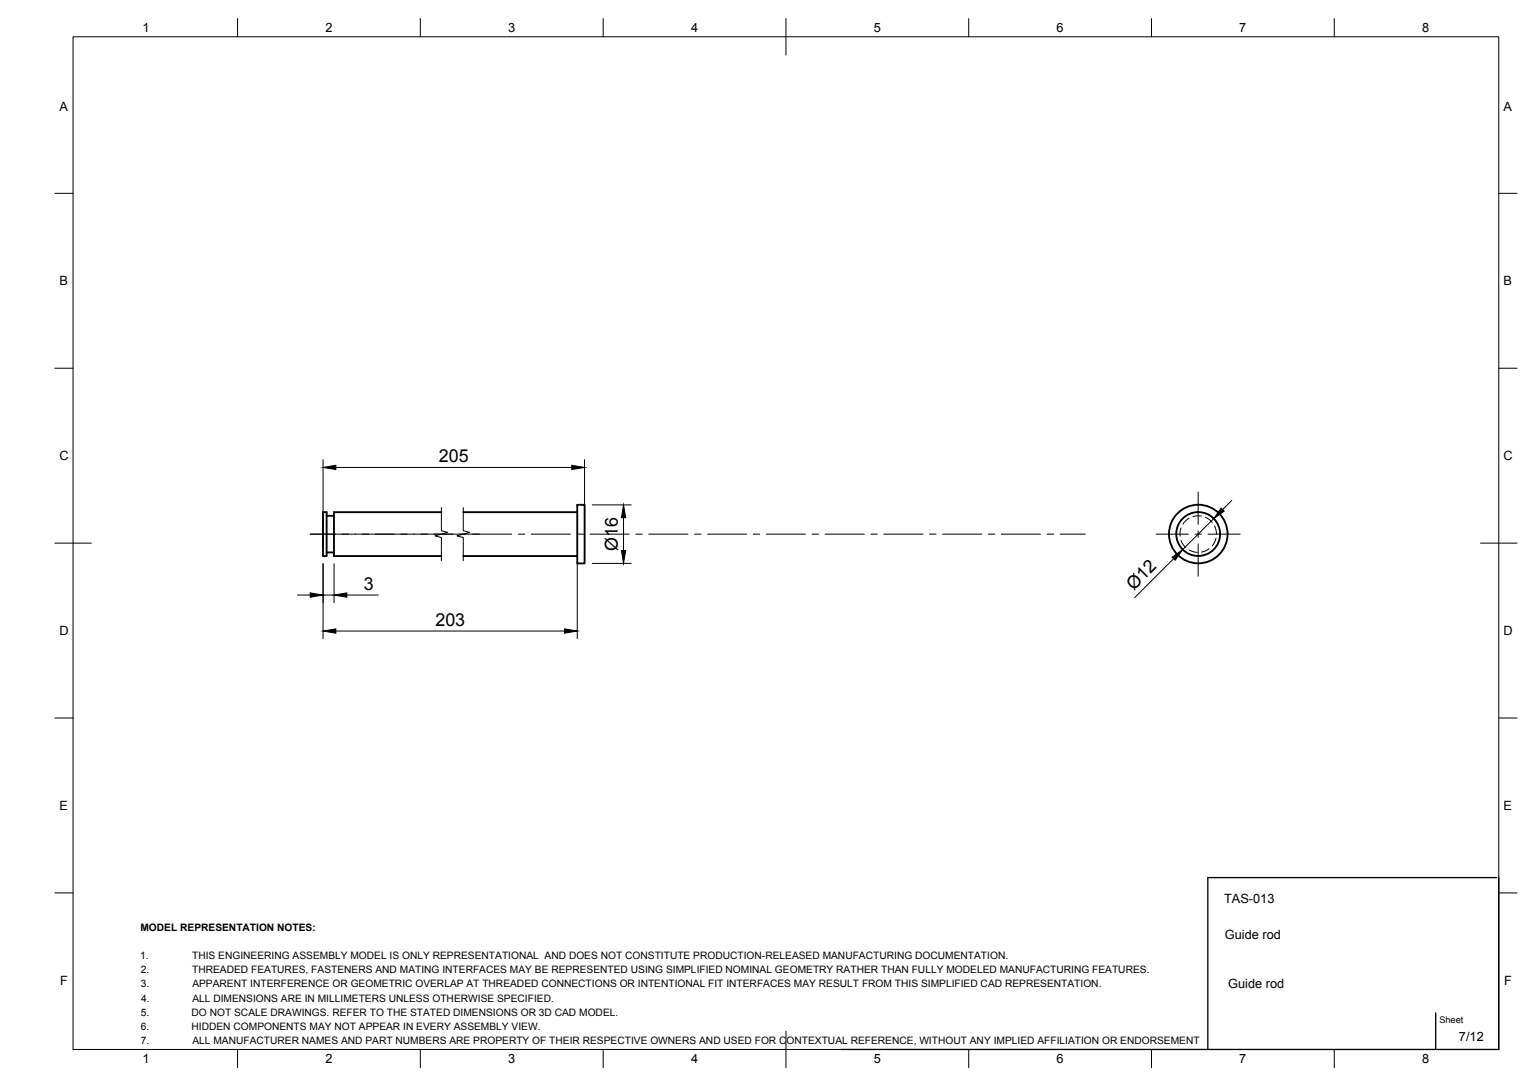
ISO-10303-21;
HEADER;
/* Generated by software containing ST-Developer
 * from STEP Tools, Inc. (www.steptools.com) 
 */

FILE_DESCRIPTION(
/* description */ (
'Independent guided parallel-jaw bracket clamp. Two12mm guide rods, re
placeable bronze sleeves, captured swiveling spindle, replaceable jaw 
pads and modeled M16x2 screw. Native slider/revolute joints linked2mm 
per revolution. Nominal opening0..122 with initial28mm. Base and two i
dentical supports welded. Standard fits, weld details and clamp load r
equire engineering selection.'),
/* implementation_level */ '2;1');

FILE_NAME(
/* name */ 'Guide rod.step',
/* time_stamp */ '2026-11-14T09:15:44-08:00',
/* author */ (''),
/* organization */ (''),
/* preprocessor_version */ 'ST-DEVELOPER v20.2',
/* originating_system */ 'Autodesk Translation Framework v15.17.0.0',
/* authorisation */ '');

FILE_SCHEMA (('AUTOMOTIVE_DESIGN { 1 0 10303 214 3 1 1 }'));
ENDSEC;

DATA;
#10=MECHANICAL_DESIGN_GEOMETRIC_PRESENTATION_REPRESENTATION('',(#922),#105806);
#898=SHAPE_REPRESENTATION_RELATIONSHIP('SRR','None',#105866,#910);
#910=ADVANCED_BREP_SHAPE_REPRESENTATION('',(#934),#105801);
#922=STYLED_ITEM('',(#105928),#934);
#934=MANIFOLD_SOLID_BREP('Body1',#7209);
#989=FACE_BOUND('',#1598,.T.);
#990=FACE_BOUND('',#1600,.T.);
#991=FACE_BOUND('',#1603,.T.);
#1042=PLANE('',#7633);
#1043=PLANE('',#7635);
#1044=PLANE('',#7639);
#1045=PLANE('',#7644);
#1046=PLANE('',#7646);
#1274=FACE_OUTER_BOUND('',#1596,.T.);
#1275=FACE_OUTER_BOUND('',#1597,.T.);
#1276=FACE_OUTER_BOUND('',#1599,.T.);
#1277=FACE_OUTER_BOUND('',#1601,.T.);
#1278=FACE_OUTER_BOUND('',#1602,.T.);
#1279=FACE_OUTER_BOUND('',#1604,.T.);
#1280=FACE_OUTER_BOUND('',#1605,.T.);
#1281=FACE_OUTER_BOUND('',#1606,.T.);
#1282=FACE_OUTER_BOUND('',#1607,.T.);
#1596=EDGE_LOOP('',(#6293,#6294,#6295,#6296));
#1597=EDGE_LOOP('',(#6297));
#1598=EDGE_LOOP('',(#6298));
#1599=EDGE_LOOP('',(#6299));
#1600=EDGE_LOOP('',(#6300));
#1601=EDGE_LOOP('',(#6301,#6302,#6303,#6304));
#1602=EDGE_LOOP('',(#6305));
#1603=EDGE_LOOP('',(#6306));
#1604=EDGE_LOOP('',(#6307,#6308,#6309,#6310));
#1605=EDGE_LOOP('',(#6311));
#1606=EDGE_LOOP('',(#6312,#6313,#6314,#6315));
#1607=EDGE_LOOP('',(#6316));
#1888=LINE('',#88770,#2168);
#1889=LINE('',#88781,#2169);
#1890=LINE('',#88789,#2170);
#1891=LINE('',#88793,#2171);
#2168=VECTOR('',#8533,5.);
#2169=VECTOR('',#8548,6.);
#2170=VECTOR('',#8557,8.);
#2171=VECTOR('',#8564,6.);
#2299=CIRCLE('',#7631,5.);
#2300=CIRCLE('',#7632,5.);
#2301=CIRCLE('',#7634,6.);
#2302=CIRCLE('',#7636,6.);
#2303=CIRCLE('',#7638,6.);
#2304=CIRCLE('',#7640,8.);
#2305=CIRCLE('',#7641,6.);
#2306=CIRCLE('',#7643,8.);
#3077=VERTEX_POINT('',#88767);
#3078=VERTEX_POINT('',#88769);
#3079=VERTEX_POINT('',#88773);
#3080=VERTEX_POINT('',#88776);
#3081=VERTEX_POINT('',#88779);
#3082=VERTEX_POINT('',#88783);
#3083=VERTEX_POINT('',#88785);
#3084=VERTEX_POINT('',#88788);
#4191=EDGE_CURVE('',#3077,#3077,#2299,.T.);
#4192=EDGE_CURVE('',#3077,#3078,#1888,.T.);
#4193=EDGE_CURVE('',#3078,#3078,#2300,.T.);
#4194=EDGE_CURVE('',#3079,#3079,#2301,.T.);
#4195=EDGE_CURVE('',#3080,#3080,#2302,.T.);
#4196=EDGE_CURVE('',#3081,#3081,#2303,.T.);
#4197=EDGE_CURVE('',#3081,#3080,#1889,.T.);
#4198=EDGE_CURVE('',#3082,#3082,#2304,.T.);
#4199=EDGE_CURVE('',#3083,#3083,#2305,.T.);
#4200=EDGE_CURVE('',#3082,#3084,#1890,.T.);
#4201=EDGE_CURVE('',#3084,#3084,#2306,.T.);
#4202=EDGE_CURVE('',#3079,#3083,#1891,.T.);
#6293=ORIENTED_EDGE('',*,*,#4191,.F.);
#6294=ORIENTED_EDGE('',*,*,#4192,.T.);
#6295=ORIENTED_EDGE('',*,*,#4193,.T.);
#6296=ORIENTED_EDGE('',*,*,#4192,.F.);
#6297=ORIENTED_EDGE('',*,*,#4194,.F.);
#6298=ORIENTED_EDGE('',*,*,#4193,.F.);
#6299=ORIENTED_EDGE('',*,*,#4195,.F.);
#6300=ORIENTED_EDGE('',*,*,#4191,.T.);
#6301=ORIENTED_EDGE('',*,*,#4196,.F.);
#6302=ORIENTED_EDGE('',*,*,#4197,.T.);
#6303=ORIENTED_EDGE('',*,*,#4195,.T.);
#6304=ORIENTED_EDGE('',*,*,#4197,.F.);
#6305=ORIENTED_EDGE('',*,*,#4198,.T.);
#6306=ORIENTED_EDGE('',*,*,#4199,.F.);
#6307=ORIENTED_EDGE('',*,*,#4198,.F.);
#6308=ORIENTED_EDGE('',*,*,#4200,.T.);
#6309=ORIENTED_EDGE('',*,*,#4201,.T.);
#6310=ORIENTED_EDGE('',*,*,#4200,.F.);
#6311=ORIENTED_EDGE('',*,*,#4201,.F.);
#6312=ORIENTED_EDGE('',*,*,#4194,.T.);
#6313=ORIENTED_EDGE('',*,*,#4202,.T.);
#6314=ORIENTED_EDGE('',*,*,#4199,.T.);
#6315=ORIENTED_EDGE('',*,*,#4202,.F.);
#6316=ORIENTED_EDGE('',*,*,#4196,.T.);
#6893=CYLINDRICAL_SURFACE('',#7630,5.);
#6894=CYLINDRICAL_SURFACE('',#7637,6.);
#6895=CYLINDRICAL_SURFACE('',#7642,8.);
#6896=CYLINDRICAL_SURFACE('',#7645,6.);
#7139=ADVANCED_FACE('',(#1274),#6893,.T.);
#7140=ADVANCED_FACE('',(#1275,#989),#1042,.F.);
#7141=ADVANCED_FACE('',(#1276,#990),#1043,.F.);
#7142=ADVANCED_FACE('',(#1277),#6894,.T.);
#7143=ADVANCED_FACE('',(#1278,#991),#1044,.T.);
#7144=ADVANCED_FACE('',(#1279),#6895,.T.);
#7145=ADVANCED_FACE('',(#1280),#1045,.F.);
#7146=ADVANCED_FACE('',(#1281),#6896,.T.);
#7147=ADVANCED_FACE('',(#1282),#1046,.T.);
#7209=CLOSED_SHELL('',(#7139,#7140,#7141,#7142,#7143,#7144,#7145,#7146,
#7147));
#7629=AXIS2_PLACEMENT_3D('',#88765,#8527,#8528);
#7630=AXIS2_PLACEMENT_3D('',#88766,#8529,#8530);
#7631=AXIS2_PLACEMENT_3D('',#88768,#8531,#8532);
#7632=AXIS2_PLACEMENT_3D('',#88771,#8534,#8535);
#7633=AXIS2_PLACEMENT_3D('',#88772,#8536,#8537);
#7634=AXIS2_PLACEMENT_3D('',#88774,#8538,#8539);
#7635=AXIS2_PLACEMENT_3D('',#88775,#8540,#8541);
#7636=AXIS2_PLACEMENT_3D('',#88777,#8542,#8543);
#7637=AXIS2_PLACEMENT_3D('',#88778,#8544,#8545);
#7638=AXIS2_PLACEMENT_3D('',#88780,#8546,#8547);
#7639=AXIS2_PLACEMENT_3D('',#88782,#8549,#8550);
#7640=AXIS2_PLACEMENT_3D('',#88784,#8551,#8552);
#7641=AXIS2_PLACEMENT_3D('',#88786,#8553,#8554);
#7642=AXIS2_PLACEMENT_3D('',#88787,#8555,#8556);
#7643=AXIS2_PLACEMENT_3D('',#88790,#8558,#8559);
#7644=AXIS2_PLACEMENT_3D('',#88791,#8560,#8561);
#7645=AXIS2_PLACEMENT_3D('',#88792,#8562,#8563);
#7646=AXIS2_PLACEMENT_3D('',#88794,#8565,#8566);
#8527=DIRECTION('axis',(0.,0.,1.));
#8528=DIRECTION('refdir',(1.,0.,0.));
#8529=DIRECTION('center_axis',(0.,0.,1.));
#8530=DIRECTION('ref_axis',(1.,0.,0.));
#8531=DIRECTION('center_axis',(0.,0.,1.));
#8532=DIRECTION('ref_axis',(1.,0.,0.));
#8533=DIRECTION('',(0.,0.,-1.));
#8534=DIRECTION('center_axis',(0.,0.,1.));
#8535=DIRECTION('ref_axis',(1.,0.,0.));
#8536=DIRECTION('center_axis',(0.,0.,-1.));
#8537=DIRECTION('ref_axis',(-1.,0.,0.));
#8538=DIRECTION('center_axis',(0.,0.,-1.));
#8539=DIRECTION('ref_axis',(1.,0.,0.));
#8540=DIRECTION('center_axis',(0.,0.,1.));
#8541=DIRECTION('ref_axis',(1.,0.,0.));
#8542=DIRECTION('center_axis',(0.,0.,1.));
#8543=DIRECTION('ref_axis',(1.,0.,0.));
#8544=DIRECTION('center_axis',(0.,0.,1.));
#8545=DIRECTION('ref_axis',(1.,0.,0.));
#8546=DIRECTION('center_axis',(0.,0.,1.));
#8547=DIRECTION('ref_axis',(1.,0.,0.));
#8548=DIRECTION('',(0.,0.,-1.));
#8549=DIRECTION('center_axis',(0.,0.,1.));
#8550=DIRECTION('ref_axis',(1.,0.,0.));
#8551=DIRECTION('center_axis',(0.,0.,1.));
#8552=DIRECTION('ref_axis',(1.,0.,0.));
#8553=DIRECTION('center_axis',(0.,0.,1.));
#8554=DIRECTION('ref_axis',(1.,0.,0.));
#8555=DIRECTION('center_axis',(0.,0.,1.));
#8556=DIRECTION('ref_axis',(1.,0.,0.));
#8557=DIRECTION('',(0.,0.,-1.));
#8558=DIRECTION('center_axis',(0.,0.,1.));
#8559=DIRECTION('ref_axis',(1.,0.,0.));
#8560=DIRECTION('center_axis',(0.,0.,1.));
#8561=DIRECTION('ref_axis',(1.,0.,0.));
#8562=DIRECTION('center_axis',(0.,0.,1.));
#8563=DIRECTION('ref_axis',(1.,0.,0.));
#8564=DIRECTION('',(0.,0.,-1.));
#8565=DIRECTION('center_axis',(0.,0.,1.));
#8566=DIRECTION('ref_axis',(1.,0.,0.));
#88765=CARTESIAN_POINT('',(0.,0.,0.));
#88766=CARTESIAN_POINT('Origin',(0.,0.,201.));
#88767=CARTESIAN_POINT('',(-5.,-6.12323399573677E-16,202.));
#88768=CARTESIAN_POINT('Origin',(0.,0.,202.));
#88769=CARTESIAN_POINT('',(-5.,-6.12323399573677E-16,200.));
#88770=CARTESIAN_POINT('',(-5.,-6.12323399573677E-16,201.));
#88771=CARTESIAN_POINT('Origin',(0.,0.,200.));
#88772=CARTESIAN_POINT('Origin',(9.,0.,200.));
#88773=CARTESIAN_POINT('',(-6.,7.34788079488412E-16,200.));
#88774=CARTESIAN_POINT('Origin',(0.,0.,200.));
#88775=CARTESIAN_POINT('Origin',(5.,0.,202.));
#88776=CARTESIAN_POINT('',(-6.,-7.34788079488412E-16,202.));
#88777=CARTESIAN_POINT('Origin',(0.,0.,202.));
#88778=CARTESIAN_POINT('Origin',(0.,0.,0.));
#88779=CARTESIAN_POINT('',(-6.,-7.34788079488412E-16,203.));
#88780=CARTESIAN_POINT('Origin',(0.,0.,203.));
#88781=CARTESIAN_POINT('',(-6.,-7.34788079488412E-16,0.));
#88782=CARTESIAN_POINT('Origin',(0.,0.,0.));
#88783=CARTESIAN_POINT('',(-8.,-9.79717439317883E-16,0.));
#88784=CARTESIAN_POINT('Origin',(0.,0.,0.));
#88785=CARTESIAN_POINT('',(-6.,-7.34788079488412E-16,0.));
#88786=CARTESIAN_POINT('Origin',(0.,0.,0.));
#88787=CARTESIAN_POINT('Origin',(0.,0.,-2.));
#88788=CARTESIAN_POINT('',(-8.,-9.79717439317883E-16,-2.));
#88789=CARTESIAN_POINT('',(-8.,-9.79717439317883E-16,-2.));
#88790=CARTESIAN_POINT('Origin',(0.,0.,-2.));
#88791=CARTESIAN_POINT('Origin',(0.,0.,-2.));
#88792=CARTESIAN_POINT('Origin',(0.,0.,0.));
#88793=CARTESIAN_POINT('',(-6.,-7.34788079488412E-16,0.));
#88794=CARTESIAN_POINT('Origin',(0.,0.,203.));
#105787=UNCERTAINTY_MEASURE_WITH_UNIT(LENGTH_MEASURE(0.01),#105807,
'DISTANCE_ACCURACY_VALUE',
'Maximum model space distance between geometric entities at asserted c
onnectivities');
#105792=UNCERTAINTY_MEASURE_WITH_UNIT(LENGTH_MEASURE(0.01),#105807,
'DISTANCE_ACCURACY_VALUE',
'Maximum model space distance between geometric entities at asserted c
onnectivities');
#105801=(
GEOMETRIC_REPRESENTATION_CONTEXT(3)
GLOBAL_UNCERTAINTY_ASSIGNED_CONTEXT((#105787))
GLOBAL_UNIT_ASSIGNED_CONTEXT((#105807,#105809,#105810))
REPRESENTATION_CONTEXT('','3D')
);
#105806=(
GEOMETRIC_REPRESENTATION_CONTEXT(3)
GLOBAL_UNCERTAINTY_ASSIGNED_CONTEXT((#105792))
GLOBAL_UNIT_ASSIGNED_CONTEXT((#105807,#105809,#105810))
REPRESENTATION_CONTEXT('','3D')
);
#105807=(
LENGTH_UNIT()
NAMED_UNIT(*)
SI_UNIT(.MILLI.,.METRE.)
);
#105809=(
NAMED_UNIT(*)
PLANE_ANGLE_UNIT()
SI_UNIT($,.RADIAN.)
);
#105810=(
NAMED_UNIT(*)
SI_UNIT($,.STERADIAN.)
SOLID_ANGLE_UNIT()
);
#105819=SHAPE_DEFINITION_REPRESENTATION(#105832,#105866);
#105832=PRODUCT_DEFINITION_SHAPE('',$,#105880);
#105866=SHAPE_REPRESENTATION('',(#7629),#105801);
#105871=PRODUCT_DEFINITION_CONTEXT('part definition',#105912,'design');
#105880=PRODUCT_DEFINITION('Guide rod','Guide rod',#105893,#105871);
#105893=PRODUCT_DEFINITION_FORMATION('',$,#105922);
#105912=APPLICATION_CONTEXT(
'Core Data for Automotive Mechanical Design Process');
#105913=PRODUCT_CONTEXT('part definition',#105912,'mechanical');
#105922=PRODUCT('Guide rod','Guide rod',$,(#105913));
#105928=PRESENTATION_STYLE_ASSIGNMENT((#105934));
#105934=SURFACE_STYLE_USAGE(.BOTH.,#105940);
#105940=SURFACE_SIDE_STYLE('',(#105946));
#105946=SURFACE_STYLE_FILL_AREA(#105952);
#105952=FILL_AREA_STYLE('Opaque(104,114,127)',(#105958));
#105958=FILL_AREA_STYLE_COLOUR('Opaque(104,114,127)',#105964);
#105964=COLOUR_RGB('Opaque(104,114,127)',0.407843137254902,0.447058823529412,
0.498039215686275);
ENDSEC;
END-ISO-10303-21;
